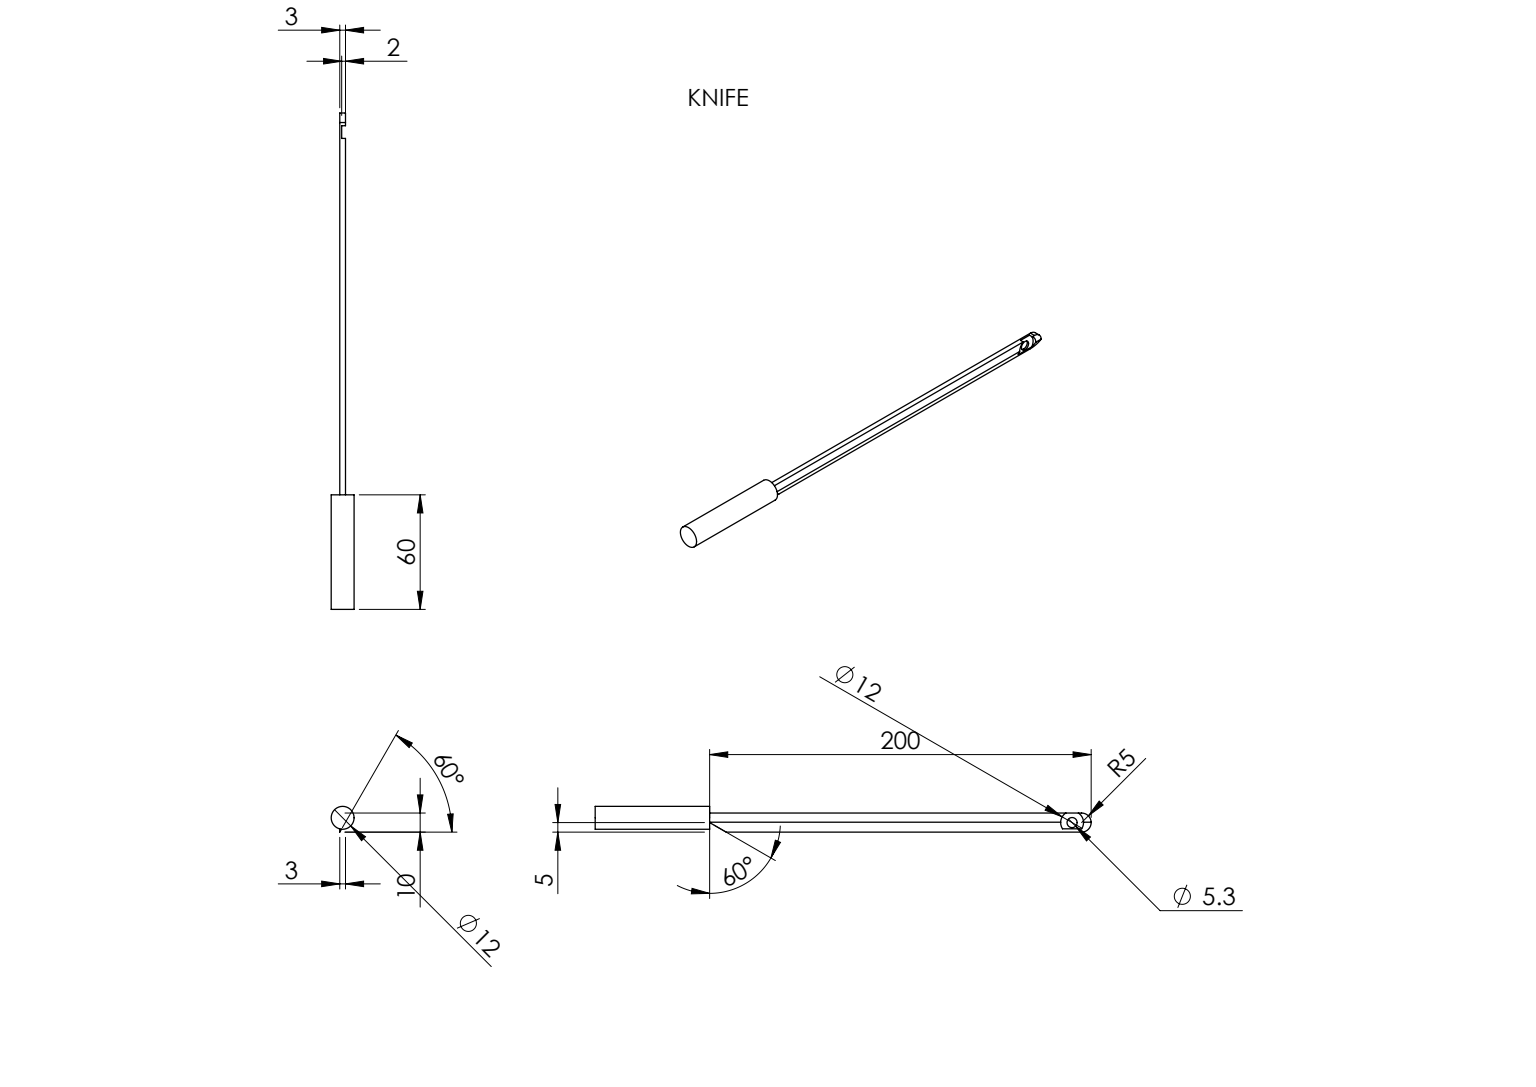
ISO-10303-21;
HEADER;
FILE_DESCRIPTION (('STEP AP214'),
    '1' );
FILE_NAME ('knife.step',
    '2026-10-25T17:17:34',
    ( '' ),
    ( '' ),
    'SwSTEP 2.0',
    'SolidWorks 2026',
    '' );
FILE_SCHEMA (( 'AUTOMOTIVE_DESIGN' ));
ENDSEC;

DATA;
#37=ORIENTED_EDGE ( 'NONE', *, *, #1725, .T. ) ;
#59=ORIENTED_EDGE ( 'NONE', *, *, #2774, .T. ) ;
#89=DIRECTION ( 'NONE',  ( 1.201851678989726239E-15, 0.8660254037844380415, -0.5000000000000009992 ) ) ;
#198=VERTEX_POINT ( 'NONE', #5871 ) ;
#209=FACE_OUTER_BOUND ( 'NONE', #12612, .T. ) ;
#217=EDGE_CURVE ( 'NONE', #4443, #15882, #16415, .T. ) ;
#255=ADVANCED_FACE ( 'NONE', ( #14648 ), #17592, .T. ) ;
#260=CIRCLE ( 'NONE', #11165, 5.000000000000000000 ) ;
#278=DIRECTION ( 'NONE',  ( 0.000000000000000000, -1.000000000000000000, 0.000000000000000000 ) ) ;
#279=ORIENTED_EDGE ( 'NONE', *, *, #11777, .T. ) ;
#382=DIRECTION ( 'NONE',  ( -1.000000000000000000, 1.387778780781445676E-15, 2.407412430484046130E-31 ) ) ;
#405=AXIS2_PLACEMENT_3D ( 'NONE', #11450, #17508, #17414 ) ;
#444=DIRECTION ( 'NONE',  ( 0.5000000000000015543, 0.8660254037844378194, 0.000000000000000000 ) ) ;
#477=DIRECTION ( 'NONE',  ( -2.775557561562891351E-15, -1.000000000000000000, 0.000000000000000000 ) ) ;
#498=MECHANICAL_DESIGN_GEOMETRIC_PRESENTATION_REPRESENTATION('',(#12637),#1099);
#504=LINE ( 'NONE', #18569, #3508 ) ;
#514=ORIENTED_EDGE ( 'NONE', *, *, #17717, .T. ) ;
#550=ADVANCED_FACE ( 'NONE', ( #16147 ), #10184, .T. ) ;
#572=VECTOR ( 'NONE', #4858, 1000.000000000000000 ) ;
#574=LINE ( 'NONE', #7790, #4310 ) ;
#577=CARTESIAN_POINT ( 'NONE',  ( 105.5000000000000142, 12.69999999999998508, 110.0000000000000142 ) ) ;
#597=ORIENTED_EDGE ( 'NONE', *, *, #11394, .T. ) ;
#600=CIRCLE ( 'NONE', #3071, 2.649999999999980371 ) ;
#617=ORIENTED_EDGE ( 'NONE', *, *, #15683, .T. ) ;
#673=DIRECTION ( 'NONE',  ( 1.000000000000000000, -1.387778780781445676E-15, -2.407412430484046130E-31 ) ) ;
#677=VERTEX_POINT ( 'NONE', #10287 ) ;
#711=VERTEX_POINT ( 'NONE', #7829 ) ;
#715=EDGE_LOOP ( 'NONE', ( #13037, #16003, #5872 ) ) ;
#728=LINE ( 'NONE', #14088, #8969 ) ;
#769=DIRECTION ( 'NONE',  ( 1.000000000000000000, -1.387778780781445676E-15, -2.407412430484046130E-31 ) ) ;
#787=DIRECTION ( 'NONE',  ( -1.000000000000000000, 1.387778780781445478E-15, 2.407412430484046130E-31 ) ) ;
#809=( LENGTH_UNIT ( ) NAMED_UNIT ( * ) SI_UNIT ( .MILLI., .METRE. ) );
#833=CIRCLE ( 'NONE', #11436, 6.000000000000015987 ) ;
#836=CARTESIAN_POINT ( 'NONE',  ( 113.0000000000000000, 10.39615242270649276, -145.9967928284264076 ) ) ;
#843=ORIENTED_EDGE ( 'NONE', *, *, #17616, .T. ) ;
#868=DIRECTION ( 'NONE',  ( -1.000000000000000000, 1.387778780781445676E-15, 2.407412430484046130E-31 ) ) ;
#894=AXIS2_PLACEMENT_3D ( 'NONE', #15497, #16581, #278 ) ;
#943=DIRECTION ( 'NONE',  ( 1.000000000000000000, -1.387778780781445676E-15, -2.407412430484046130E-31 ) ) ;
#1045=CARTESIAN_POINT ( 'NONE',  ( 113.0000000000000142, 15.19999999999997442, -150.0000000000000000 ) ) ;
#1083=EDGE_LOOP ( 'NONE', ( #7928, #14869 ) ) ;
#1099=( GEOMETRIC_REPRESENTATION_CONTEXT ( 3 ) GLOBAL_UNCERTAINTY_ASSIGNED_CONTEXT ( ( #7539 ) ) GLOBAL_UNIT_ASSIGNED_CONTEXT ( ( #809, #14267, #11443 ) ) REPRESENTATION_CONTEXT ( 'NONE', 'WORKASPACE' ) );
#1103=CARTESIAN_POINT ( 'NONE',  ( 110.0000000000000568, 5.199999999999976197, -150.0000000000000000 ) ) ;
#1113=CARTESIAN_POINT ( 'NONE',  ( 111.5987303322250597, 7.969082163015147380, -145.7054384624938166 ) ) ;
#1232=CARTESIAN_POINT ( 'NONE',  ( 110.0000000000000000, 10.19999999999997620, -142.6499999999999773 ) ) ;
#1257=EDGE_CURVE ( 'NONE', #4300, #18769, #504, .T. ) ;
#1302=DIRECTION ( 'NONE',  ( 1.000000000000000000, -1.387778780781445676E-15, -2.407412430484046130E-31 ) ) ;
#1322=EDGE_LOOP ( 'NONE', ( #17514, #16605, #7351, #5363, #8386 ) ) ;
#1333=DIRECTION ( 'NONE',  ( -1.387778780781445478E-15, -1.000000000000000000, -1.214306433183764966E-16 ) ) ;
#1353=ORIENTED_EDGE ( 'NONE', *, *, #4995, .T. ) ;
#1384=LINE ( 'NONE', #3919, #4252 ) ;
#1445=CIRCLE ( 'NONE', #16413, 6.000000000000015987 ) ;
#1446=CARTESIAN_POINT ( 'NONE',  ( 109.9999999999999716, -14.00063509461108247, 8.083270440699362069 ) ) ;
#1454=CARTESIAN_POINT ( 'NONE',  ( 111.0000000000000000, 10.19999999999997620, -139.9999999999999716 ) ) ;
#1562=ORIENTED_EDGE ( 'NONE', *, *, #6040, .T. ) ;
#1604=EDGE_CURVE ( 'NONE', #5913, #4731, #14539, .T. ) ;
#1630=AXIS2_PLACEMENT_3D ( 'NONE', #8981, #4593, #2930 ) ;
#1665=VERTEX_POINT ( 'NONE', #14443 ) ;
#1672=FACE_BOUND ( 'NONE', #5012, .T. ) ;
#1719=DIRECTION ( 'NONE',  ( 7.222237291452147586E-32, -1.214306433183764966E-16, 1.000000000000000000 ) ) ;
#1725=EDGE_CURVE ( 'NONE', #4443, #17789, #10375, .T. ) ;
#1741=ORIENTED_EDGE ( 'NONE', *, *, #7576, .F. ) ;
#1759=EDGE_CURVE ( 'NONE', #4731, #17788, #9431, .T. ) ;
#1776=VERTEX_POINT ( 'NONE', #11380 ) ;
#1833=CARTESIAN_POINT ( 'NONE',  ( 111.0000000000000000, 15.19999999999997620, -143.3166247903554336 ) ) ;
#1930=AXIS2_PLACEMENT_3D ( 'NONE', #14747, #4304, #7423 ) ;
#2056=CIRCLE ( 'NONE', #7671, 2.649999999999985700 ) ;
#2158=PRESENTATION_STYLE_ASSIGNMENT (( #9576 ) ) ;
#2179=DIRECTION ( 'NONE',  ( -1.000000000000000000, 1.387778780781445478E-15, 2.407412430484046130E-31 ) ) ;
#2240=DIRECTION ( 'NONE',  ( 1.000000000000000000, -1.387778780781445676E-15, -2.407412430484046130E-31 ) ) ;
#2265=EDGE_CURVE ( 'NONE', #711, #15407, #14092, .T. ) ;
#2336=PLANE ( 'NONE',  #16751 ) ;
#2342=( LENGTH_UNIT ( ) NAMED_UNIT ( * ) SI_UNIT ( .MILLI., .METRE. ) );
#2409=DIRECTION ( 'NONE',  ( 1.387778780781445676E-15, 1.000000000000000000, 0.000000000000000000 ) ) ;
#2423=ORIENTED_EDGE ( 'NONE', *, *, #9224, .F. ) ;
#2453=VECTOR ( 'NONE', #673, 1000.000000000000000 ) ;
#2476=DIRECTION ( 'NONE',  ( -7.222237291452147586E-32, 1.214306433183764966E-16, -1.000000000000000000 ) ) ;
#2493=PRODUCT ( 'knife', 'knife', '', ( #12777 ) ) ;
#2535=CARTESIAN_POINT ( 'NONE',  ( 113.0000000000000000, 10.39615242270649276, -134.0032071715735640 ) ) ;
#2558=DIRECTION ( 'NONE',  ( -7.222237291452147586E-32, 1.214306433183764966E-16, -1.000000000000000000 ) ) ;
#2594=DIRECTION ( 'NONE',  ( 2.312964634635736745E-15, 1.000000000000000000, 0.000000000000000000 ) ) ;
#2599=PLANE ( 'NONE',  #2724 ) ;
#2643=CARTESIAN_POINT ( 'NONE',  ( 111.0000000000000000, 10.19999999999997620, -139.9999999999999716 ) ) ;
#2698=ORIENTED_EDGE ( 'NONE', *, *, #15683, .F. ) ;
#2724=AXIS2_PLACEMENT_3D ( 'NONE', #15994, #17559, #6920 ) ;
#2738=VERTEX_POINT ( 'NONE', #18288 ) ;
#2750=CYLINDRICAL_SURFACE ( 'NONE', #7410, 2.649999999999985700 ) ;
#2760=DIRECTION ( 'NONE',  ( 0.8660254037844378194, -0.5000000000000015543, -6.071532165918849482E-17 ) ) ;
#2772=PLANE ( 'NONE',  #11462 ) ;
#2774=EDGE_CURVE ( 'NONE', #15407, #14034, #5192, .T. ) ;
#2839=CARTESIAN_POINT ( 'NONE',  ( 113.0000000000000000, 10.19999999999997264, -139.9999999999999716 ) ) ;
#2848=DIRECTION ( 'NONE',  ( 1.000000000000000000, -0.000000000000000000, -2.407412430484046130E-31 ) ) ;
#2909=CIRCLE ( 'NONE', #13819, 6.000000000000005329 ) ;
#2930=DIRECTION ( 'NONE',  ( 2.312964634635736745E-15, 1.000000000000000000, 0.000000000000000000 ) ) ;
#2964=ORIENTED_EDGE ( 'NONE', *, *, #6872, .F. ) ;
#2981=DIRECTION ( 'NONE',  ( 0.000000000000000000, 0.000000000000000000, 1.000000000000000000 ) ) ;
#3021=CARTESIAN_POINT ( 'NONE',  ( 111.0000000000000142, 15.19999999999997797, -136.6833752096445380 ) ) ;
#3031=EDGE_CURVE ( 'NONE', #6366, #14034, #13631, .T. ) ;
#3054=AXIS2_PLACEMENT_3D ( 'NONE', #12607, #15347, #17107 ) ;
#3071=AXIS2_PLACEMENT_3D ( 'NONE', #13290, #10083, #16040 ) ;
#3191=DIRECTION ( 'NONE',  ( 2.407412430484046130E-31, -3.340955887615246502E-46, 1.000000000000000000 ) ) ;
#3223=DIRECTION ( 'NONE',  ( -1.000000000000000000, 1.387778780781445676E-15, 2.407412430484046130E-31 ) ) ;
#3227=EDGE_LOOP ( 'NONE', ( #15134, #19037 ) ) ;
#3292=LINE ( 'NONE', #577, #8679 ) ;
#3334=DIRECTION ( 'NONE',  ( 1.000000000000000000, 0.000000000000000000, 0.000000000000000000 ) ) ;
#3336=VECTOR ( 'NONE', #11034, 1000.000000000000000 ) ;
#3363=AXIS2_PLACEMENT_3D ( 'NONE', #17741, #10592, #17636 ) ;
#3462=( BOUNDED_CURVE ( )  B_SPLINE_CURVE ( 3, ( #2535, #18583, #14359, #5396 ),
 .UNSPECIFIED., .F., .F. ) 
 B_SPLINE_CURVE_WITH_KNOTS ( ( 4, 4 ),
 ( 1.538098430149248408, 2.146777830243033147 ),
 .UNSPECIFIED. ) 
 CURVE ( )  GEOMETRIC_REPRESENTATION_ITEM ( )  RATIONAL_B_SPLINE_CURVE ( ( 1.000000000000000000, 0.9693633521240627715, 0.9693633521240627715, 1.000000000000000000 ) ) 
 REPRESENTATION_ITEM ( '' )  );
#3482=CARTESIAN_POINT ( 'NONE',  ( 111.0000000000000000, 6.932050807568743700, -145.0319487353994532 ) ) ;
#3485=LINE ( 'NONE', #1833, #2453 ) ;
#3508=VECTOR ( 'NONE', #8111, 1000.000000000000000 ) ;
#3528=UNCERTAINTY_MEASURE_WITH_UNIT (LENGTH_MEASURE( 1.000000000000000082E-05 ), #13971, 'distance_accuracy_value', 'NONE');
#3586=CARTESIAN_POINT ( 'NONE',  ( 111.1957315586905537, 7.271067811865449926, -150.0000000000000000 ) ) ;
#3635=AXIS2_PLACEMENT_3D ( 'NONE', #7880, #7786, #3191 ) ;
#3711=EDGE_LOOP ( 'NONE', ( #3889, #17571, #13602, #7033 ) ) ;
#3777=CARTESIAN_POINT ( 'NONE',  ( 110.0000000000000000, 5.199999999999952216, 50.00000000000001421 ) ) ;
#3781=DIRECTION ( 'NONE',  ( -2.775557561562891351E-15, -1.000000000000000000, 0.000000000000000000 ) ) ;
#3816=ORIENTED_EDGE ( 'NONE', *, *, #11616, .F. ) ;
#3876=CARTESIAN_POINT ( 'NONE',  ( 110.0000000000000000, 5.199999999999975309, -145.0000000000000000 ) ) ;
#3888=LINE ( 'NONE', #8570, #14101 ) ;
#3889=ORIENTED_EDGE ( 'NONE', *, *, #9772, .F. ) ;
#3919=CARTESIAN_POINT ( 'NONE',  ( 111.0000000000000000, 6.932050807568743700, -150.0000000000000000 ) ) ;
#3925=EDGE_CURVE ( 'NONE', #13993, #17953, #4299, .T. ) ;
#3940=CIRCLE ( 'NONE', #9874, 6.000000000000005329 ) ;
#3950=PRODUCT_DEFINITION_FORMATION_WITH_SPECIFIED_SOURCE ( 'ANY', '', #2493, .NOT_KNOWN. ) ;
#3979=ORIENTED_EDGE ( 'NONE', *, *, #8908, .T. ) ;
#4007=CARTESIAN_POINT ( 'NONE',  ( 113.0000000000000000, 10.39615242270649453, -145.0000000000000000 ) ) ;
#4111=ORIENTED_EDGE ( 'NONE', *, *, #1604, .T. ) ;
#4141=VECTOR ( 'NONE', #6550, 1000.000000000000000 ) ;
#4142=VECTOR ( 'NONE', #9971, 1000.000000000000000 ) ;
#4202=ORIENTED_EDGE ( 'NONE', *, *, #12497, .F. ) ;
#4252=VECTOR ( 'NONE', #9885, 1000.000000000000000 ) ;
#4299=CIRCLE ( 'NONE', #8653, 6.000000000000015987 ) ;
#4300=VERTEX_POINT ( 'NONE', #18580 ) ;
#4304=DIRECTION ( 'NONE',  ( 0.000000000000000000, 0.000000000000000000, 1.000000000000000000 ) ) ;
#4308=CARTESIAN_POINT ( 'NONE',  ( 111.0000000000000000, 10.19999999999997620, -139.9999999999999716 ) ) ;
#4310=VECTOR ( 'NONE', #13744, 999.9999999999998863 ) ;
#4354=ADVANCED_FACE ( 'NONE', ( #8119 ), #18196, .T. ) ;
#4372=ORIENTED_EDGE ( 'NONE', *, *, #15167, .T. ) ;
#4396=EDGE_CURVE ( 'NONE', #4731, #15882, #16016, .T. ) ;
#4400=CYLINDRICAL_SURFACE ( 'NONE', #1630, 6.000000000000015987 ) ;
#4422=ORIENTED_EDGE ( 'NONE', *, *, #3031, .F. ) ;
#4443=VERTEX_POINT ( 'NONE', #12994 ) ;
#4467=CARTESIAN_POINT ( 'NONE',  ( 113.0000000000000000, 10.39615242270649453, -149.9961509411812415 ) ) ;
#4563=ORIENTED_EDGE ( 'NONE', *, *, #3925, .T. ) ;
#4593=DIRECTION ( 'NONE',  ( 1.000000000000000000, -1.387778780781445676E-15, -2.407412430484046130E-31 ) ) ;
#4637=ORIENTED_EDGE ( 'NONE', *, *, #1257, .F. ) ;
#4731=VERTEX_POINT ( 'NONE', #4467 ) ;
#4760=ORIENTED_EDGE ( 'NONE', *, *, #11777, .F. ) ;
#4858=DIRECTION ( 'NONE',  ( -1.000000000000000000, 1.387778780781445676E-15, 2.407412430484046130E-31 ) ) ;
#4868=ORIENTED_EDGE ( 'NONE', *, *, #14583, .F. ) ;
#4877=VERTEX_POINT ( 'NONE', #18432 ) ;
#4922=VECTOR ( 'NONE', #9580, 1000.000000000000000 ) ;
#4929=( GEOMETRIC_REPRESENTATION_CONTEXT ( 3 ) GLOBAL_UNCERTAINTY_ASSIGNED_CONTEXT ( ( #3528 ) ) GLOBAL_UNIT_ASSIGNED_CONTEXT ( ( #13971, #12894, #5290 ) ) REPRESENTATION_CONTEXT ( 'NONE', 'WORKASPACE' ) );
#4946=EDGE_CURVE ( 'NONE', #10357, #4877, #14906, .T. ) ;
#4963=FACE_OUTER_BOUND ( 'NONE', #715, .T. ) ;
#4995=EDGE_CURVE ( 'NONE', #6366, #8755, #12277, .T. ) ;
#5012=EDGE_LOOP ( 'NONE', ( #14719, #11712 ) ) ;
#5090=FACE_BOUND ( 'NONE', #1083, .T. ) ;
#5123=CARTESIAN_POINT ( 'NONE',  ( 113.6225952641917161, 11.47451905283827855, 50.00000000000001421 ) ) ;
#5182=DIRECTION ( 'NONE',  ( 1.387778780781445676E-15, 1.000000000000000000, 0.000000000000000000 ) ) ;
#5188=CARTESIAN_POINT ( 'NONE',  ( 105.5000000000000142, 12.69999999999998508, 110.0000000000000142 ) ) ;
#5192=LINE ( 'NONE', #16914, #4922 ) ;
#5267=ORIENTED_EDGE ( 'NONE', *, *, #7090, .T. ) ;
#5290=( NAMED_UNIT ( * ) SI_UNIT ( $, .STERADIAN. ) SOLID_ANGLE_UNIT ( ) );
#5363=ORIENTED_EDGE ( 'NONE', *, *, #13804, .F. ) ;
#5396=CARTESIAN_POINT ( 'NONE',  ( 111.0000000000000000, 6.932050807568741924, -134.9680512646005184 ) ) ;
#5441=VERTEX_POINT ( 'NONE', #16943 ) ;
#5442=DIRECTION ( 'NONE',  ( -2.775557561562891351E-15, -1.000000000000000000, 0.000000000000000000 ) ) ;
#5487=SURFACE_STYLE_FILL_AREA ( #15543 ) ;
#5504=CARTESIAN_POINT ( 'NONE',  ( 117.5000000000000142, 12.69999999999998508, 110.0000000000000142 ) ) ;
#5531=CARTESIAN_POINT ( 'NONE',  ( 113.0000000000000000, 10.19999999999997264, -145.0000000000000000 ) ) ;
#5702=ORIENTED_EDGE ( 'NONE', *, *, #11394, .F. ) ;
#5704=ADVANCED_FACE ( 'NONE', ( #7325 ), #4400, .F. ) ;
#5707=APPLICATION_CONTEXT ( 'automotive_design' ) ;
#5782=CARTESIAN_POINT ( 'NONE',  ( 112.8867513459481984, 10.19999999999997264, -150.0000000000000000 ) ) ;
#5787=AXIS2_PLACEMENT_3D ( 'NONE', #12206, #15328, #15237 ) ;
#5829=CARTESIAN_POINT ( 'NONE',  ( 111.0000000000000000, 10.19999999999997620, -139.9999999999999716 ) ) ;
#5871=CARTESIAN_POINT ( 'NONE',  ( 113.0000000000000000, 15.19999999999996732, -143.3166247903554336 ) ) ;
#5872=ORIENTED_EDGE ( 'NONE', *, *, #7090, .F. ) ;
#5913=VERTEX_POINT ( 'NONE', #9855 ) ;
#6040=EDGE_CURVE ( 'NONE', #17953, #8755, #3888, .T. ) ;
#6067=CARTESIAN_POINT ( 'NONE',  ( 111.5000000000000142, 12.69999999999998508, 110.0000000000000142 ) ) ;
#6079=ORIENTED_EDGE ( 'NONE', *, *, #6040, .F. ) ;
#6137=LINE ( 'NONE', #1446, #18929 ) ;
#6164=PLANE ( 'NONE',  #13877 ) ;
#6166=DIRECTION ( 'NONE',  ( 0.000000000000000000, 1.000000000000000000, 0.000000000000000000 ) ) ;
#6334=ORIENTED_EDGE ( 'NONE', *, *, #13908, .F. ) ;
#6338=CARTESIAN_POINT ( 'NONE',  ( 113.0000000000000142, 15.19999999999997442, -150.0000000000000000 ) ) ;
#6366=VERTEX_POINT ( 'NONE', #10168 ) ;
#6425=ORIENTED_EDGE ( 'NONE', *, *, #8908, .F. ) ;
#6450=DIRECTION ( 'NONE',  ( -1.000000000000000000, 1.387778780781445676E-15, 2.407412430484046130E-31 ) ) ;
#6484=VERTEX_POINT ( 'NONE', #17163 ) ;
#6550=DIRECTION ( 'NONE',  ( 1.000000000000000000, -1.387778780781445478E-15, -2.407412430484046130E-31 ) ) ;
#6610=ORIENTED_EDGE ( 'NONE', *, *, #17833, .T. ) ;
#6730=( BOUNDED_CURVE ( )  B_SPLINE_CURVE ( 3, ( #11007, #3586, #9546, #3876 ),
 .UNSPECIFIED., .F., .F. ) 
 B_SPLINE_CURVE_WITH_KNOTS ( ( 4, 4 ),
 ( 4.712388980384689674, 6.283185307179586232 ),
 .UNSPECIFIED. ) 
 CURVE ( )  GEOMETRIC_REPRESENTATION_ITEM ( )  RATIONAL_B_SPLINE_CURVE ( ( 1.000000000000000000, 0.8047378541243649375, 0.8047378541243649375, 1.000000000000000000 ) ) 
 REPRESENTATION_ITEM ( '' )  );
#6748=CARTESIAN_POINT ( 'NONE',  ( 111.0000000000000000, 10.19999999999997620, -142.6499999999999773 ) ) ;
#6755=( NAMED_UNIT ( * ) PLANE_ANGLE_UNIT ( ) SI_UNIT ( $, .RADIAN. ) );
#6872=EDGE_CURVE ( 'NONE', #15407, #1665, #17620, .T. ) ;
#6876=EDGE_LOOP ( 'NONE', ( #6079, #11959, #17666, #18967, #16129, #2698, #4422, #1353 ) ) ;
#6920=DIRECTION ( 'NONE',  ( 1.000000000000000000, 0.000000000000000000, -0.000000000000000000 ) ) ;
#6957=DIRECTION ( 'NONE',  ( 2.312964634635736745E-15, 1.000000000000000000, 0.000000000000000000 ) ) ;
#7019=DIRECTION ( 'NONE',  ( 7.222237291452147586E-32, -1.214306433183764966E-16, 1.000000000000000000 ) ) ;
#7033=ORIENTED_EDGE ( 'NONE', *, *, #6872, .T. ) ;
#7090=EDGE_CURVE ( 'NONE', #1776, #711, #18179, .T. ) ;
#7191=DIRECTION ( 'NONE',  ( 1.000000000000000000, -1.387778780781445676E-15, -2.407412430484046130E-31 ) ) ;
#7228=CARTESIAN_POINT ( 'NONE',  ( 110.0000000000000000, 5.199999999999976197, -150.0000000000000000 ) ) ;
#7239=EDGE_CURVE ( 'NONE', #17788, #4300, #9861, .T. ) ;
#7302=DIRECTION ( 'NONE',  ( 6.938893903907244155E-16, 0.5000000000000009992, 0.8660254037844380415 ) ) ;
#7325=FACE_OUTER_BOUND ( 'NONE', #19153, .T. ) ;
#7341=CARTESIAN_POINT ( 'NONE',  ( 0.000000000000000000, 0.000000000000000000, 0.000000000000000000 ) ) ;
#7344=AXIS2_PLACEMENT_3D ( 'NONE', #10524, #89, #11989 ) ;
#7351=ORIENTED_EDGE ( 'NONE', *, *, #217, .F. ) ;
#7366=( GEOMETRIC_REPRESENTATION_CONTEXT ( 3 ) GLOBAL_UNCERTAINTY_ASSIGNED_CONTEXT ( ( #8016 ) ) GLOBAL_UNIT_ASSIGNED_CONTEXT ( ( #2342, #6755, #12799 ) ) REPRESENTATION_CONTEXT ( 'NONE', 'WORKASPACE' ) );
#7407=DIRECTION ( 'NONE',  ( 0.000000000000000000, 0.000000000000000000, -1.000000000000000000 ) ) ;
#7410=AXIS2_PLACEMENT_3D ( 'NONE', #2643, #2848, #8998 ) ;
#7423=DIRECTION ( 'NONE',  ( 1.000000000000000000, 0.000000000000000000, -0.000000000000000000 ) ) ;
#7426=DIRECTION ( 'NONE',  ( 1.000000000000000000, -1.387778780781445478E-15, -2.407412430484046130E-31 ) ) ;
#7539=UNCERTAINTY_MEASURE_WITH_UNIT (LENGTH_MEASURE( 1.000000000000000082E-05 ), #809, 'distance_accuracy_value', 'NONE');
#7542=ORIENTED_EDGE ( 'NONE', *, *, #11616, .T. ) ;
#7576=EDGE_CURVE ( 'NONE', #14117, #12107, #14113, .T. ) ;
#7582=AXIS2_PLACEMENT_3D ( 'NONE', #15551, #8224, #9879 ) ;
#7671=AXIS2_PLACEMENT_3D ( 'NONE', #4308, #16033, #14652 ) ;
#7749=SHAPE_REPRESENTATION ( 'knife', ( #10540 ), #4929 ) ;
#7786=DIRECTION ( 'NONE',  ( -1.000000000000000000, 1.387778780781445676E-15, 2.407412430484046130E-31 ) ) ;
#7790=CARTESIAN_POINT ( 'NONE',  ( 110.2307692307692832, 5.599704032515842478, 42.03205365446332564 ) ) ;
#7793=CARTESIAN_POINT ( 'NONE',  ( 110.0000000000000000, 5.199999999999975309, -145.0000000000000000 ) ) ;
#7796=DIRECTION ( 'NONE',  ( 2.312964634635736745E-15, 1.000000000000000000, 0.000000000000000000 ) ) ;
#7829=CARTESIAN_POINT ( 'NONE',  ( 112.8867513459481984, 10.19999999999995310, 50.00000000000001421 ) ) ;
#7880=CARTESIAN_POINT ( 'NONE',  ( 112.9999999999999858, -1.568190022283033361E-13, -2.720376046446971763E-29 ) ) ;
#7928=ORIENTED_EDGE ( 'NONE', *, *, #12453, .F. ) ;
#7950=APPLICATION_CONTEXT ( 'automotive_design' ) ;
#7973=PLANE ( 'NONE',  #7344 ) ;
#8016=UNCERTAINTY_MEASURE_WITH_UNIT (LENGTH_MEASURE( 1.000000000000000082E-05 ), #2342, 'distance_accuracy_value', 'NONE');
#8085=DIRECTION ( 'NONE',  ( 7.222237291452147586E-32, -1.214306433183764966E-16, 1.000000000000000000 ) ) ;
#8111=DIRECTION ( 'NONE',  ( 7.222237291452147586E-32, -1.214306433183764966E-16, 1.000000000000000000 ) ) ;
#8119=FACE_OUTER_BOUND ( 'NONE', #16655, .T. ) ;
#8208=CARTESIAN_POINT ( 'NONE',  ( 111.0000000000000000, 10.19999999999997620, -139.9999999999999716 ) ) ;
#8214=SURFACE_SIDE_STYLE ('',( #5487 ) ) ;
#8224=DIRECTION ( 'NONE',  ( 0.000000000000000000, 0.000000000000000000, 1.000000000000000000 ) ) ;
#8299=LINE ( 'NONE', #6748, #3336 ) ;
#8306=ORIENTED_EDGE ( 'NONE', *, *, #8667, .F. ) ;
#8309=CARTESIAN_POINT ( 'NONE',  ( 112.9622674055505342, 10.33079765201859779, -149.9987168157428528 ) ) ;
#8386=ORIENTED_EDGE ( 'NONE', *, *, #7239, .F. ) ;
#8402=ORIENTED_EDGE ( 'NONE', *, *, #13303, .T. ) ;
#8540=ORIENTED_EDGE ( 'NONE', *, *, #12814, .T. ) ;
#8570=CARTESIAN_POINT ( 'NONE',  ( 111.0000000000000142, 15.19999999999997797, -150.0000000000000000 ) ) ;
#8647=CARTESIAN_POINT ( 'NONE',  ( 113.0000000000000142, 15.19999999999994955, 50.00000000000001421 ) ) ;
#8653=AXIS2_PLACEMENT_3D ( 'NONE', #8713, #1302, #11555 ) ;
#8667=EDGE_CURVE ( 'NONE', #12107, #14117, #14433, .T. ) ;
#8679=VECTOR ( 'NONE', #12572, 1000.000000000000000 ) ;
#8713=CARTESIAN_POINT ( 'NONE',  ( 111.0000000000000000, 10.19999999999997620, -139.9999999999999716 ) ) ;
#8740=EDGE_CURVE ( 'NONE', #1665, #6484, #3462, .T. ) ;
#8755=VERTEX_POINT ( 'NONE', #3021 ) ;
#8879=EDGE_LOOP ( 'NONE', ( #1741, #8306 ) ) ;
#8908=EDGE_CURVE ( 'NONE', #17789, #11431, #14646, .T. ) ;
#8969=VECTOR ( 'NONE', #2179, 1000.000000000000000 ) ;
#8981=CARTESIAN_POINT ( 'NONE',  ( 111.0000000000000000, 10.19999999999997620, -139.9999999999999716 ) ) ;
#8988=VECTOR ( 'NONE', #18206, 1000.000000000000000 ) ;
#8998=DIRECTION ( 'NONE',  ( 0.000000000000000000, 0.000000000000000000, -1.000000000000000000 ) ) ;
#9021=CARTESIAN_POINT ( 'NONE',  ( 113.0000000000000000, 10.19999999999997264, -145.0000000000000000 ) ) ;
#9048=CARTESIAN_POINT ( 'NONE',  ( 113.0000000000000142, 15.19999999999997442, -150.0000000000000000 ) ) ;
#9089=EDGE_LOOP ( 'NONE', ( #1562, #279, #4202, #4563 ) ) ;
#9131=CARTESIAN_POINT ( 'NONE',  ( 111.5000000000000142, 12.69999999999998508, 110.0000000000000142 ) ) ;
#9181=DIRECTION ( 'NONE',  ( 2.407412430484046130E-31, -3.340955887615246502E-46, 1.000000000000000000 ) ) ;
#9224=EDGE_CURVE ( 'NONE', #16242, #2738, #2909, .T. ) ;
#9230=PRODUCT_DEFINITION_CONTEXT ( 'detailed design', #7950, 'design' ) ;
#9362=EDGE_LOOP ( 'NONE', ( #19251, #5267, #17151, #59, #617 ) ) ;
#9400=MANIFOLD_SOLID_BREP ( 'M5 Clearance Hole1', #17271 ) ;
#9431=CIRCLE ( 'NONE', #18178, 5.000000000000000000 ) ;
#9477=ORIENTED_EDGE ( 'NONE', *, *, #4995, .F. ) ;
#9508=ADVANCED_FACE ( 'NONE', ( #17986 ), #14650, .T. ) ;
#9546=CARTESIAN_POINT ( 'NONE',  ( 110.0000000000000568, 5.199999999999975309, -147.9289321881345245 ) ) ;
#9551=SHAPE_DEFINITION_REPRESENTATION ( #17162, #7749 ) ;
#9576=SURFACE_STYLE_USAGE ( .BOTH. , #8214 ) ;
#9580=DIRECTION ( 'NONE',  ( 1.387778780781445676E-15, 1.000000000000000000, 0.000000000000000000 ) ) ;
#9603=EDGE_LOOP ( 'NONE', ( #13879, #597, #10759, #10616 ) ) ;
#9714=ADVANCED_FACE ( 'NONE', ( #209 ), #6164, .F. ) ;
#9772=EDGE_CURVE ( 'NONE', #6366, #1665, #14827, .T. ) ;
#9779=CARTESIAN_POINT ( 'NONE',  ( 112.9245130097707204, 10.26540512031890273, -150.0000000000000284 ) ) ;
#9793=LINE ( 'NONE', #5504, #12043 ) ;
#9809=FACE_OUTER_BOUND ( 'NONE', #3711, .T. ) ;
#9810=CARTESIAN_POINT ( 'NONE',  ( 112.2864669432758831, 9.160276915580402246, -146.0372177658591681 ) ) ;
#9842=AXIS2_PLACEMENT_3D ( 'NONE', #6067, #17594, #10358 ) ;
#9855=CARTESIAN_POINT ( 'NONE',  ( 113.0000000000000000, 10.39615242270649276, -145.9967928284264076 ) ) ;
#9861=LINE ( 'NONE', #17382, #15364 ) ;
#9868=EDGE_LOOP ( 'NONE', ( #10911, #2964, #12425, #6334, #6425, #15448, #16842, #16103, #5702, #17657 ) ) ;
#9870=FILL_AREA_STYLE_COLOUR ( '', #15848 ) ;
#9874=AXIS2_PLACEMENT_3D ( 'NONE', #9131, #2981, #16570 ) ;
#9879=DIRECTION ( 'NONE',  ( 1.000000000000000000, 0.000000000000000000, 0.000000000000000000 ) ) ;
#9885=DIRECTION ( 'NONE',  ( 7.222237291452149776E-32, -1.214306433183765213E-16, 1.000000000000000000 ) ) ;
#9941=AXIS2_PLACEMENT_3D ( 'NONE', #9021, #16734, #18115 ) ;
#9971=DIRECTION ( 'NONE',  ( -7.222237291452147586E-32, 1.214306433183764966E-16, -1.000000000000000000 ) ) ;
#10083=DIRECTION ( 'NONE',  ( -1.000000000000000000, 1.387778780781445676E-15, 2.407412430484046130E-31 ) ) ;
#10165=CARTESIAN_POINT ( 'NONE',  ( 113.0000000000000142, 10.19999999999997264, -150.0000000000000000 ) ) ;
#10168=CARTESIAN_POINT ( 'NONE',  ( 113.0000000000000000, 15.19999999999996732, -136.6833752096445380 ) ) ;
#10180=ADVANCED_FACE ( 'NONE', ( #4963 ), #7973, .F. ) ;
#10184=PLANE ( 'NONE',  #17227 ) ;
#10287=CARTESIAN_POINT ( 'NONE',  ( 111.0000000000000000, 10.19999999999997620, -142.6499999999999773 ) ) ;
#10357=VERTEX_POINT ( 'NONE', #1232 ) ;
#10358=DIRECTION ( 'NONE',  ( -1.000000000000000000, 0.000000000000000000, 0.000000000000000000 ) ) ;
#10375=CIRCLE ( 'NONE', #16308, 5.000000000000000000 ) ;
#10461=CARTESIAN_POINT ( 'NONE',  ( 110.0000000000000142, 15.19999999999995310, 50.00000000000001421 ) ) ;
#10480=ADVANCED_FACE ( 'NONE', ( #13333 ), #14695, .F. ) ;
#10524=CARTESIAN_POINT ( 'NONE',  ( 113.0000000000000000, 5.199999999999948663, 41.33974596215564645 ) ) ;
#10540=AXIS2_PLACEMENT_3D ( 'NONE', #7341, #19270, #11738 ) ;
#10569=VECTOR ( 'NONE', #2409, 1000.000000000000000 ) ;
#10592=DIRECTION ( 'NONE',  ( 1.000000000000000000, -0.000000000000000000, -2.407412430484046130E-31 ) ) ;
#10616=ORIENTED_EDGE ( 'NONE', *, *, #17770, .F. ) ;
#10664=DIRECTION ( 'NONE',  ( 0.000000000000000000, 0.000000000000000000, 1.000000000000000000 ) ) ;
#10759=ORIENTED_EDGE ( 'NONE', *, *, #12466, .T. ) ;
#10816=CARTESIAN_POINT ( 'NONE',  ( 111.0000000000000142, 15.19999999999997797, -143.3166247903554336 ) ) ;
#10860=CARTESIAN_POINT ( 'NONE',  ( 111.5000000000000142, 12.69999999999998508, 110.0000000000000142 ) ) ;
#10888=CARTESIAN_POINT ( 'NONE',  ( 117.5000000000000142, 12.69999999999998508, 50.00000000000001421 ) ) ;
#10911=ORIENTED_EDGE ( 'NONE', *, *, #8740, .F. ) ;
#11007=CARTESIAN_POINT ( 'NONE',  ( 112.8867513459481984, 10.19999999999997264, -150.0000000000000000 ) ) ;
#11028=CARTESIAN_POINT ( 'NONE',  ( 113.0000000000000142, 10.19999999999995310, 50.00000000000001421 ) ) ;
#11034=DIRECTION ( 'NONE',  ( 1.000000000000000000, -0.000000000000000000, -2.407412430484046130E-31 ) ) ;
#11165=AXIS2_PLACEMENT_3D ( 'NONE', #18155, #382, #477 ) ;
#11211=FACE_BOUND ( 'NONE', #9362, .T. ) ;
#11380=CARTESIAN_POINT ( 'NONE',  ( 110.0000000000000142, 10.19999999999995666, 50.00000000000001421 ) ) ;
#11394=EDGE_CURVE ( 'NONE', #13993, #5913, #13297, .T. ) ;
#11431=VERTEX_POINT ( 'NONE', #18901 ) ;
#11436=AXIS2_PLACEMENT_3D ( 'NONE', #5829, #7191, #2594 ) ;
#11443=( NAMED_UNIT ( * ) SI_UNIT ( $, .STERADIAN. ) SOLID_ANGLE_UNIT ( ) );
#11450=CARTESIAN_POINT ( 'NONE',  ( 111.5000000000000142, 12.69999999999998508, 50.00000000000001421 ) ) ;
#11456=VECTOR ( 'NONE', #1719, 1000.000000000000000 ) ;
#11462=AXIS2_PLACEMENT_3D ( 'NONE', #13577, #3223, #9181 ) ;
#11555=DIRECTION ( 'NONE',  ( 2.312964634635736745E-15, 1.000000000000000000, 0.000000000000000000 ) ) ;
#11616=EDGE_CURVE ( 'NONE', #2738, #12107, #9793, .T. ) ;
#11712=ORIENTED_EDGE ( 'NONE', *, *, #18566, .F. ) ;
#11738=DIRECTION ( 'NONE',  ( 1.000000000000000000, 0.000000000000000000, 0.000000000000000000 ) ) ;
#11777=EDGE_CURVE ( 'NONE', #8755, #6484, #833, .T. ) ;
#11782=CARTESIAN_POINT ( 'NONE',  ( 113.0000000000000142, 10.39615242270647144, 50.00000000000001421 ) ) ;
#11913=PRODUCT_DEFINITION ( 'UNKNOWN', '', #3950, #9230 ) ;
#11959=ORIENTED_EDGE ( 'NONE', *, *, #17770, .T. ) ;
#11980=EDGE_CURVE ( 'NONE', #2738, #16242, #3940, .T. ) ;
#11989=DIRECTION ( 'NONE',  ( -1.000000000000000000, 1.387778780781445478E-15, 2.407412430484046130E-31 ) ) ;
#12041=CARTESIAN_POINT ( 'NONE',  ( 111.0000000000000000, 10.19999999999997620, -137.3499999999999943 ) ) ;
#12043=VECTOR ( 'NONE', #17509, 1000.000000000000000 ) ;
#12107=VERTEX_POINT ( 'NONE', #10888 ) ;
#12113=CARTESIAN_POINT ( 'NONE',  ( 112.9999999999999858, -1.568190022283033361E-13, -2.720376046446971763E-29 ) ) ;
#12206=CARTESIAN_POINT ( 'NONE',  ( 113.0000000000000000, 10.19999999999997264, -139.9999999999999716 ) ) ;
#12277=LINE ( 'NONE', #18240, #572 ) ;
#12365=AXIS2_PLACEMENT_3D ( 'NONE', #18086, #7426, #6166 ) ;
#12401=DIRECTION ( 'NONE',  ( 2.407412430484046130E-31, -3.340955887615246502E-46, 1.000000000000000000 ) ) ;
#12425=ORIENTED_EDGE ( 'NONE', *, *, #2265, .F. ) ;
#12453=EDGE_CURVE ( 'NONE', #677, #5441, #2056, .T. ) ;
#12466=EDGE_CURVE ( 'NONE', #5913, #198, #1445, .T. ) ;
#12480=FACE_OUTER_BOUND ( 'NONE', #9603, .T. ) ;
#12488=EDGE_LOOP ( 'NONE', ( #16955, #18267, #15615, #15643 ) ) ;
#12497=EDGE_CURVE ( 'NONE', #13993, #6484, #1384, .T. ) ;
#12562=ADVANCED_FACE ( 'NONE', ( #16704 ), #13673, .T. ) ;
#12572=DIRECTION ( 'NONE',  ( -0.000000000000000000, -0.000000000000000000, -1.000000000000000000 ) ) ;
#12607=CARTESIAN_POINT ( 'NONE',  ( 111.5000000000000142, 12.69999999999998508, 110.0000000000000142 ) ) ;
#12612=EDGE_LOOP ( 'NONE', ( #14306, #4111, #13181, #6610 ) ) ;
#12637=STYLED_ITEM('',(#19378),#9400);
#12777=PRODUCT_CONTEXT ( 'NONE', #5707, 'mechanical' ) ;
#12799=( NAMED_UNIT ( * ) SI_UNIT ( $, .STERADIAN. ) SOLID_ANGLE_UNIT ( ) );
#12814=EDGE_CURVE ( 'NONE', #11431, #1776, #6137, .T. ) ;
#12894=( NAMED_UNIT ( * ) PLANE_ANGLE_UNIT ( ) SI_UNIT ( $, .RADIAN. ) );
#12930=ADVANCED_FACE ( 'NONE', ( #9809 ), #18344, .F. ) ;
#12994=CARTESIAN_POINT ( 'NONE',  ( 110.0000000000000000, 10.19999999999997620, -150.0000000000000000 ) ) ;
#13037=ORIENTED_EDGE ( 'NONE', *, *, #12814, .F. ) ;
#13114=ORIENTED_EDGE ( 'NONE', *, *, #18924, .T. ) ;
#13181=ORIENTED_EDGE ( 'NONE', *, *, #1759, .T. ) ;
#13191=DIRECTION ( 'NONE',  ( 1.000000000000000000, -1.387778780781445676E-15, -2.407412430484046130E-31 ) ) ;
#13213=CARTESIAN_POINT ( 'NONE',  ( 113.0000000000000000, 10.39615242270649453, -145.0000000000000000 ) ) ;
#13290=CARTESIAN_POINT ( 'NONE',  ( 110.0000000000000000, 10.19999999999997620, -139.9999999999999716 ) ) ;
#13293=FACE_OUTER_BOUND ( 'NONE', #19305, .T. ) ;
#13297=( BOUNDED_CURVE ( )  B_SPLINE_CURVE ( 3, ( #14388, #1113, #9810, #836 ),
 .UNSPECIFIED., .F., .F. ) 
 B_SPLINE_CURVE_WITH_KNOTS ( ( 4, 4 ),
 ( 4.136407476936552641, 4.745086877030337824 ),
 .UNSPECIFIED. ) 
 CURVE ( )  GEOMETRIC_REPRESENTATION_ITEM ( )  RATIONAL_B_SPLINE_CURVE ( ( 1.000000000000000000, 0.9693633521240625495, 0.9693633521240625495, 1.000000000000000000 ) ) 
 REPRESENTATION_ITEM ( '' )  );
#13303=EDGE_CURVE ( 'NONE', #4877, #5441, #15163, .T. ) ;
#13316=VECTOR ( 'NONE', #444, 999.9999999999998863 ) ;
#13333=FACE_OUTER_BOUND ( 'NONE', #6876, .T. ) ;
#13506=VECTOR ( 'NONE', #19155, 1000.000000000000000 ) ;
#13517=FACE_OUTER_BOUND ( 'NONE', #12488, .T. ) ;
#13577=CARTESIAN_POINT ( 'NONE',  ( 109.9999999999999858, -1.526556658859589991E-13, -2.648153673532450419E-29 ) ) ;
#13602=ORIENTED_EDGE ( 'NONE', *, *, #2774, .F. ) ;
#13631=LINE ( 'NONE', #9048, #11456 ) ;
#13673=CYLINDRICAL_SURFACE ( 'NONE', #12365, 5.000000000000000888 ) ;
#13744=DIRECTION ( 'NONE',  ( 0.2773500981126160725, 0.4803844614152618653, 0.8320502943378429439 ) ) ;
#13804=EDGE_CURVE ( 'NONE', #4300, #4443, #260, .T. ) ;
#13819=AXIS2_PLACEMENT_3D ( 'NONE', #10860, #10664, #3334 ) ;
#13877=AXIS2_PLACEMENT_3D ( 'NONE', #12113, #6450, #12401 ) ;
#13879=ORIENTED_EDGE ( 'NONE', *, *, #3925, .F. ) ;
#13908=EDGE_CURVE ( 'NONE', #11431, #711, #574, .T. ) ;
#13962=AXIS2_PLACEMENT_3D ( 'NONE', #18354, #769, #7796 ) ;
#13965=STYLED_ITEM ( 'NONE', ( #2158 ), #16702 ) ;
#13971=( LENGTH_UNIT ( ) NAMED_UNIT ( * ) SI_UNIT ( .MILLI., .METRE. ) );
#13979=AXIS2_PLACEMENT_3D ( 'NONE', #1454, #14934, #7407 ) ;
#13993=VERTEX_POINT ( 'NONE', #3482 ) ;
#14034=VERTEX_POINT ( 'NONE', #8647 ) ;
#14088=CARTESIAN_POINT ( 'NONE',  ( 113.0000000000000142, 15.19999999999994955, 50.00000000000001421 ) ) ;
#14092=LINE ( 'NONE', #5123, #13316 ) ;
#14101=VECTOR ( 'NONE', #7019, 1000.000000000000000 ) ;
#14113=CIRCLE ( 'NONE', #405, 6.000000000000005329 ) ;
#14117=VERTEX_POINT ( 'NONE', #18833 ) ;
#14267=( NAMED_UNIT ( * ) PLANE_ANGLE_UNIT ( ) SI_UNIT ( $, .RADIAN. ) );
#14306=ORIENTED_EDGE ( 'NONE', *, *, #12466, .F. ) ;
#14359=CARTESIAN_POINT ( 'NONE',  ( 111.5987303322250597, 7.969082163015149156, -134.2945615375061550 ) ) ;
#14388=CARTESIAN_POINT ( 'NONE',  ( 111.0000000000000000, 6.932050807568743700, -145.0319487353994532 ) ) ;
#14417=FACE_OUTER_BOUND ( 'NONE', #8879, .T. ) ;
#14433=CIRCLE ( 'NONE', #7582, 6.000000000000005329 ) ;
#14443=CARTESIAN_POINT ( 'NONE',  ( 113.0000000000000000, 10.39615242270649276, -134.0032071715735640 ) ) ;
#14474=ADVANCED_FACE ( 'NONE', ( #1672, #16161 ), #2772, .T. ) ;
#14539=LINE ( 'NONE', #4007, #4142 ) ;
#14543=CARTESIAN_POINT ( 'NONE',  ( 113.0000000000000000, 10.39615242270649453, -149.9961509411812415 ) ) ;
#14583=EDGE_CURVE ( 'NONE', #10357, #677, #8299, .T. ) ;
#14599=ADVANCED_FACE ( 'NONE', ( #5090, #18279 ), #2336, .T. ) ;
#14646=LINE ( 'NONE', #7228, #13506 ) ;
#14648=FACE_OUTER_BOUND ( 'NONE', #3227, .T. ) ;
#14650=CYLINDRICAL_SURFACE ( 'NONE', #9842, 6.000000000000005329 ) ;
#14652=DIRECTION ( 'NONE',  ( 0.000000000000000000, 0.000000000000000000, -1.000000000000000000 ) ) ;
#14695=PLANE ( 'NONE',  #18596 ) ;
#14719=ORIENTED_EDGE ( 'NONE', *, *, #4946, .F. ) ;
#14741=ORIENTED_EDGE ( 'NONE', *, *, #11980, .F. ) ;
#14747=CARTESIAN_POINT ( 'NONE',  ( 111.5000000000000142, 12.69999999999998508, 110.0000000000000142 ) ) ;
#14827=CIRCLE ( 'NONE', #5787, 6.000000000000015987 ) ;
#14869=ORIENTED_EDGE ( 'NONE', *, *, #17616, .F. ) ;
#14906=CIRCLE ( 'NONE', #894, 2.649999999999980371 ) ;
#14934=DIRECTION ( 'NONE',  ( 1.000000000000000000, -0.000000000000000000, -2.407412430484046130E-31 ) ) ;
#15063=EDGE_LOOP ( 'NONE', ( #14741, #7542, #17374, #16317 ) ) ;
#15120=LINE ( 'NONE', #6338, #17111 ) ;
#15134=ORIENTED_EDGE ( 'NONE', *, *, #9224, .T. ) ;
#15163=LINE ( 'NONE', #12041, #8988 ) ;
#15167=EDGE_CURVE ( 'NONE', #15882, #17789, #6730, .T. ) ;
#15237=DIRECTION ( 'NONE',  ( 2.312964634635736745E-15, 1.000000000000000000, 0.000000000000000000 ) ) ;
#15328=DIRECTION ( 'NONE',  ( 1.000000000000000000, -1.387778780781445676E-15, -2.407412430484046130E-31 ) ) ;
#15347=DIRECTION ( 'NONE',  ( -0.000000000000000000, -0.000000000000000000, -1.000000000000000000 ) ) ;
#15362=FACE_OUTER_BOUND ( 'NONE', #16202, .T. ) ;
#15364=VECTOR ( 'NONE', #787, 1000.000000000000000 ) ;
#15407=VERTEX_POINT ( 'NONE', #11782 ) ;
#15411=CARTESIAN_POINT ( 'NONE',  ( 113.0000000000000142, 15.19999999999997442, -145.0000000000000000 ) ) ;
#15448=ORIENTED_EDGE ( 'NONE', *, *, #15167, .F. ) ;
#15497=CARTESIAN_POINT ( 'NONE',  ( 110.0000000000000000, 10.19999999999997620, -139.9999999999999716 ) ) ;
#15543=FILL_AREA_STYLE ('',( #9870 ) ) ;
#15551=CARTESIAN_POINT ( 'NONE',  ( 111.5000000000000142, 12.69999999999998508, 50.00000000000001421 ) ) ;
#15615=ORIENTED_EDGE ( 'NONE', *, *, #14583, .T. ) ;
#15623=ORIENTED_EDGE ( 'NONE', *, *, #8740, .T. ) ;
#15643=ORIENTED_EDGE ( 'NONE', *, *, #12453, .T. ) ;
#15683=EDGE_CURVE ( 'NONE', #14034, #18769, #728, .T. ) ;
#15713=CARTESIAN_POINT ( 'NONE',  ( 110.0000000000000000, 10.19999999999997620, -145.0000000000000000 ) ) ;
#15848=COLOUR_RGB ( '',0.8941176470588234615, 0.8941176470588234615, 0.8941176470588234615 ) ;
#15851=ADVANCED_FACE ( 'NONE', ( #13293 ), #2750, .F. ) ;
#15882=VERTEX_POINT ( 'NONE', #5782 ) ;
#15944=ADVANCED_FACE ( 'NONE', ( #12480 ), #18543, .F. ) ;
#15994=CARTESIAN_POINT ( 'NONE',  ( 111.5000000000000142, 12.69999999999998508, 50.00000000000001421 ) ) ;
#16003=ORIENTED_EDGE ( 'NONE', *, *, #13908, .T. ) ;
#16016=( BOUNDED_CURVE ( )  B_SPLINE_CURVE ( 3, ( #14543, #8309, #9779, #17496 ),
 .UNSPECIFIED., .F., .F. ) 
 B_SPLINE_CURVE_WITH_KNOTS ( ( 4, 4 ),
 ( 1.531555772456618891, 1.570796326794896780 ),
 .UNSPECIFIED. ) 
 CURVE ( )  GEOMETRIC_REPRESENTATION_ITEM ( )  RATIONAL_B_SPLINE_CURVE ( ( 1.000000000000000000, 0.9998716856909537487, 0.9998716856909537487, 1.000000000000000000 ) ) 
 REPRESENTATION_ITEM ( '' )  );
#16033=DIRECTION ( 'NONE',  ( 1.000000000000000000, -0.000000000000000000, -2.407412430484046130E-31 ) ) ;
#16040=DIRECTION ( 'NONE',  ( 0.000000000000000000, -1.000000000000000000, 0.000000000000000000 ) ) ;
#16103=ORIENTED_EDGE ( 'NONE', *, *, #1604, .F. ) ;
#16117=MECHANICAL_DESIGN_GEOMETRIC_PRESENTATION_REPRESENTATION('',(#13965),#7366);
#16129=ORIENTED_EDGE ( 'NONE', *, *, #1257, .T. ) ;
#16147=FACE_OUTER_BOUND ( 'NONE', #9868, .T. ) ;
#16161=FACE_OUTER_BOUND ( 'NONE', #18643, .T. ) ;
#16184=ADVANCED_FACE ( 'NONE', ( #11211, #14417 ), #2599, .F. ) ;
#16202=EDGE_LOOP ( 'NONE', ( #16439, #4372, #18170 ) ) ;
#16242=VERTEX_POINT ( 'NONE', #5188 ) ;
#16289=VECTOR ( 'NONE', #17690, 1000.000000000000000 ) ;
#16307=VECTOR ( 'NONE', #2476, 1000.000000000000000 ) ;
#16308=AXIS2_PLACEMENT_3D ( 'NONE', #15713, #868, #3781 ) ;
#16317=ORIENTED_EDGE ( 'NONE', *, *, #17717, .F. ) ;
#16385=ORIENTED_EDGE ( 'NONE', *, *, #7576, .T. ) ;
#16413=AXIS2_PLACEMENT_3D ( 'NONE', #2839, #13191, #6957 ) ;
#16415=LINE ( 'NONE', #10165, #16289 ) ;
#16439=ORIENTED_EDGE ( 'NONE', *, *, #217, .T. ) ;
#16570=DIRECTION ( 'NONE',  ( 1.000000000000000000, 0.000000000000000000, 0.000000000000000000 ) ) ;
#16581=DIRECTION ( 'NONE',  ( -1.000000000000000000, 1.387778780781445676E-15, 2.407412430484046130E-31 ) ) ;
#16605=ORIENTED_EDGE ( 'NONE', *, *, #4396, .T. ) ;
#16655=EDGE_LOOP ( 'NONE', ( #3816, #2423, #514, #16385 ) ) ;
#16702=ADVANCED_BREP_SHAPE_REPRESENTATION ( '', ( #9400, #10540 ), #4929 ) ;
#16704=FACE_OUTER_BOUND ( 'NONE', #1322, .T. ) ;
#16734=DIRECTION ( 'NONE',  ( -1.000000000000000000, 1.387778780781445478E-15, 2.407412430484046130E-31 ) ) ;
#16751=AXIS2_PLACEMENT_3D ( 'NONE', #8208, #2240, #5182 ) ;
#16842=ORIENTED_EDGE ( 'NONE', *, *, #4396, .F. ) ;
#16910=SHAPE_REPRESENTATION_RELATIONSHIP ( 'NONE' , 'NONE' ,  #7749, #16702 ) ;
#16914=CARTESIAN_POINT ( 'NONE',  ( 113.0000000000000000, 5.199999999999947775, 50.00000000000001421 ) ) ;
#16943=CARTESIAN_POINT ( 'NONE',  ( 111.0000000000000000, 10.19999999999997620, -137.3499999999999943 ) ) ;
#16955=ORIENTED_EDGE ( 'NONE', *, *, #13303, .F. ) ;
#17001=ADVANCED_FACE ( 'NONE', ( #13517 ), #17828, .F. ) ;
#17107=DIRECTION ( 'NONE',  ( -1.000000000000000000, 0.000000000000000000, 0.000000000000000000 ) ) ;
#17111=VECTOR ( 'NONE', #8085, 1000.000000000000000 ) ;
#17151=ORIENTED_EDGE ( 'NONE', *, *, #2265, .T. ) ;
#17162=PRODUCT_DEFINITION_SHAPE ( 'NONE', 'NONE',  #11913 ) ;
#17163=CARTESIAN_POINT ( 'NONE',  ( 111.0000000000000000, 6.932050807568741924, -134.9680512646005184 ) ) ;
#17174=LINE ( 'NONE', #3777, #10569 ) ;
#17227=AXIS2_PLACEMENT_3D ( 'NONE', #1103, #2760, #2558 ) ;
#17271=CLOSED_SHELL ( 'NONE', ( #15851, #9508, #12930, #9714, #10480, #14474, #10180, #12562, #18242, #4354, #255, #16184, #550, #15944, #5704, #14599, #17001 ) ) ;
#17374=ORIENTED_EDGE ( 'NONE', *, *, #8667, .T. ) ;
#17382=CARTESIAN_POINT ( 'NONE',  ( 110.0000000000000142, 15.19999999999997797, -145.0000000000000000 ) ) ;
#17414=DIRECTION ( 'NONE',  ( 1.000000000000000000, 0.000000000000000000, 0.000000000000000000 ) ) ;
#17423=CIRCLE ( 'NONE', #13979, 2.649999999999985700 ) ;
#17451=ORIENTED_EDGE ( 'NONE', *, *, #4946, .T. ) ;
#17496=CARTESIAN_POINT ( 'NONE',  ( 112.8867513459481984, 10.19999999999997264, -150.0000000000000000 ) ) ;
#17508=DIRECTION ( 'NONE',  ( 0.000000000000000000, 0.000000000000000000, 1.000000000000000000 ) ) ;
#17509=DIRECTION ( 'NONE',  ( -0.000000000000000000, -0.000000000000000000, -1.000000000000000000 ) ) ;
#17514=ORIENTED_EDGE ( 'NONE', *, *, #1759, .F. ) ;
#17559=DIRECTION ( 'NONE',  ( 0.000000000000000000, 0.000000000000000000, 1.000000000000000000 ) ) ;
#17571=ORIENTED_EDGE ( 'NONE', *, *, #3031, .T. ) ;
#17592=PLANE ( 'NONE',  #1930 ) ;
#17594=DIRECTION ( 'NONE',  ( -0.000000000000000000, -0.000000000000000000, -1.000000000000000000 ) ) ;
#17616=EDGE_CURVE ( 'NONE', #5441, #677, #17423, .T. ) ;
#17620=LINE ( 'NONE', #13213, #16307 ) ;
#17636=DIRECTION ( 'NONE',  ( 0.000000000000000000, 0.000000000000000000, -1.000000000000000000 ) ) ;
#17657=ORIENTED_EDGE ( 'NONE', *, *, #12497, .T. ) ;
#17666=ORIENTED_EDGE ( 'NONE', *, *, #17833, .F. ) ;
#17690=DIRECTION ( 'NONE',  ( 1.000000000000000000, -1.387778780781445478E-15, -2.407412430484046130E-31 ) ) ;
#17717=EDGE_CURVE ( 'NONE', #16242, #14117, #3292, .T. ) ;
#17741=CARTESIAN_POINT ( 'NONE',  ( 111.0000000000000000, 10.19999999999997620, -139.9999999999999716 ) ) ;
#17770=EDGE_CURVE ( 'NONE', #17953, #198, #3485, .T. ) ;
#17783=ORIENTED_EDGE ( 'NONE', *, *, #9772, .T. ) ;
#17788=VERTEX_POINT ( 'NONE', #15411 ) ;
#17789=VERTEX_POINT ( 'NONE', #7793 ) ;
#17828=CYLINDRICAL_SURFACE ( 'NONE', #3363, 2.649999999999985700 ) ;
#17833=EDGE_CURVE ( 'NONE', #17788, #198, #15120, .T. ) ;
#17953=VERTEX_POINT ( 'NONE', #10816 ) ;
#17986=FACE_OUTER_BOUND ( 'NONE', #15063, .T. ) ;
#18021=CYLINDRICAL_SURFACE ( 'NONE', #9941, 5.000000000000000000 ) ;
#18086=CARTESIAN_POINT ( 'NONE',  ( 113.0000000000000142, 10.19999999999997264, -145.0000000000000000 ) ) ;
#18115=DIRECTION ( 'NONE',  ( 0.000000000000000000, -1.000000000000000000, 0.000000000000000000 ) ) ;
#18155=CARTESIAN_POINT ( 'NONE',  ( 110.0000000000000000, 10.19999999999997620, -145.0000000000000000 ) ) ;
#18170=ORIENTED_EDGE ( 'NONE', *, *, #1725, .F. ) ;
#18178=AXIS2_PLACEMENT_3D ( 'NONE', #5531, #943, #5442 ) ;
#18179=LINE ( 'NONE', #11028, #4141 ) ;
#18196=CYLINDRICAL_SURFACE ( 'NONE', #3054, 6.000000000000005329 ) ;
#18206=DIRECTION ( 'NONE',  ( 1.000000000000000000, -0.000000000000000000, -2.407412430484046130E-31 ) ) ;
#18222=ORIENTED_EDGE ( 'NONE', *, *, #13804, .T. ) ;
#18240=CARTESIAN_POINT ( 'NONE',  ( 111.0000000000000000, 15.19999999999997620, -136.6833752096445380 ) ) ;
#18242=ADVANCED_FACE ( 'NONE', ( #15362 ), #18021, .T. ) ;
#18267=ORIENTED_EDGE ( 'NONE', *, *, #18566, .T. ) ;
#18279=FACE_OUTER_BOUND ( 'NONE', #9089, .T. ) ;
#18288=CARTESIAN_POINT ( 'NONE',  ( 117.5000000000000142, 12.69999999999998508, 110.0000000000000142 ) ) ;
#18344=PLANE ( 'NONE',  #3635 ) ;
#18354=CARTESIAN_POINT ( 'NONE',  ( 111.0000000000000000, 10.19999999999997620, -139.9999999999999716 ) ) ;
#18432=CARTESIAN_POINT ( 'NONE',  ( 110.0000000000000000, 10.19999999999997620, -137.3499999999999943 ) ) ;
#18543=CYLINDRICAL_SURFACE ( 'NONE', #13962, 6.000000000000015987 ) ;
#18566=EDGE_CURVE ( 'NONE', #4877, #10357, #600, .T. ) ;
#18569=CARTESIAN_POINT ( 'NONE',  ( 110.0000000000000142, 15.19999999999997797, -150.0000000000000000 ) ) ;
#18580=CARTESIAN_POINT ( 'NONE',  ( 110.0000000000000142, 15.19999999999997797, -145.0000000000000000 ) ) ;
#18583=CARTESIAN_POINT ( 'NONE',  ( 112.2864669432758831, 9.160276915580404022, -133.9627822341408034 ) ) ;
#18596=AXIS2_PLACEMENT_3D ( 'NONE', #1045, #1333, #19017 ) ;
#18643=EDGE_LOOP ( 'NONE', ( #18222, #37, #3979, #8540, #13114, #4637 ) ) ;
#18769=VERTEX_POINT ( 'NONE', #10461 ) ;
#18833=CARTESIAN_POINT ( 'NONE',  ( 105.5000000000000142, 12.69999999999998508, 50.00000000000001421 ) ) ;
#18901=CARTESIAN_POINT ( 'NONE',  ( 110.0000000000000000, 5.199999999999953104, 41.33974596215564645 ) ) ;
#18924=EDGE_CURVE ( 'NONE', #1776, #18769, #17174, .T. ) ;
#18929=VECTOR ( 'NONE', #7302, 1000.000000000000000 ) ;
#18967=ORIENTED_EDGE ( 'NONE', *, *, #7239, .T. ) ;
#19017=DIRECTION ( 'NONE',  ( 1.000000000000000000, -1.387778780781445478E-15, 0.000000000000000000 ) ) ;
#19037=ORIENTED_EDGE ( 'NONE', *, *, #11980, .T. ) ;
#19153=EDGE_LOOP ( 'NONE', ( #17783, #15623, #4760, #9477 ) ) ;
#19155=DIRECTION ( 'NONE',  ( 7.222237291452147586E-32, -1.214306433183764966E-16, 1.000000000000000000 ) ) ;
#19251=ORIENTED_EDGE ( 'NONE', *, *, #18924, .F. ) ;
#19270=DIRECTION ( 'NONE',  ( 0.000000000000000000, 0.000000000000000000, 1.000000000000000000 ) ) ;
#19305=EDGE_LOOP ( 'NONE', ( #17451, #8402, #843, #4868 ) ) ;
#19372=COLOUR_RGB('Off White',0.89,0.88,0.83);
#19373=FILL_AREA_STYLE_COLOUR('',#19372);
#19374=FILL_AREA_STYLE('',(#19373));
#19375=SURFACE_STYLE_FILL_AREA(#19374);
#19376=SURFACE_SIDE_STYLE('',(#19375));
#19377=SURFACE_STYLE_USAGE(.BOTH.,#19376);
#19378=PRESENTATION_STYLE_ASSIGNMENT((#19377));
ENDSEC;
END-ISO-10303-21;
